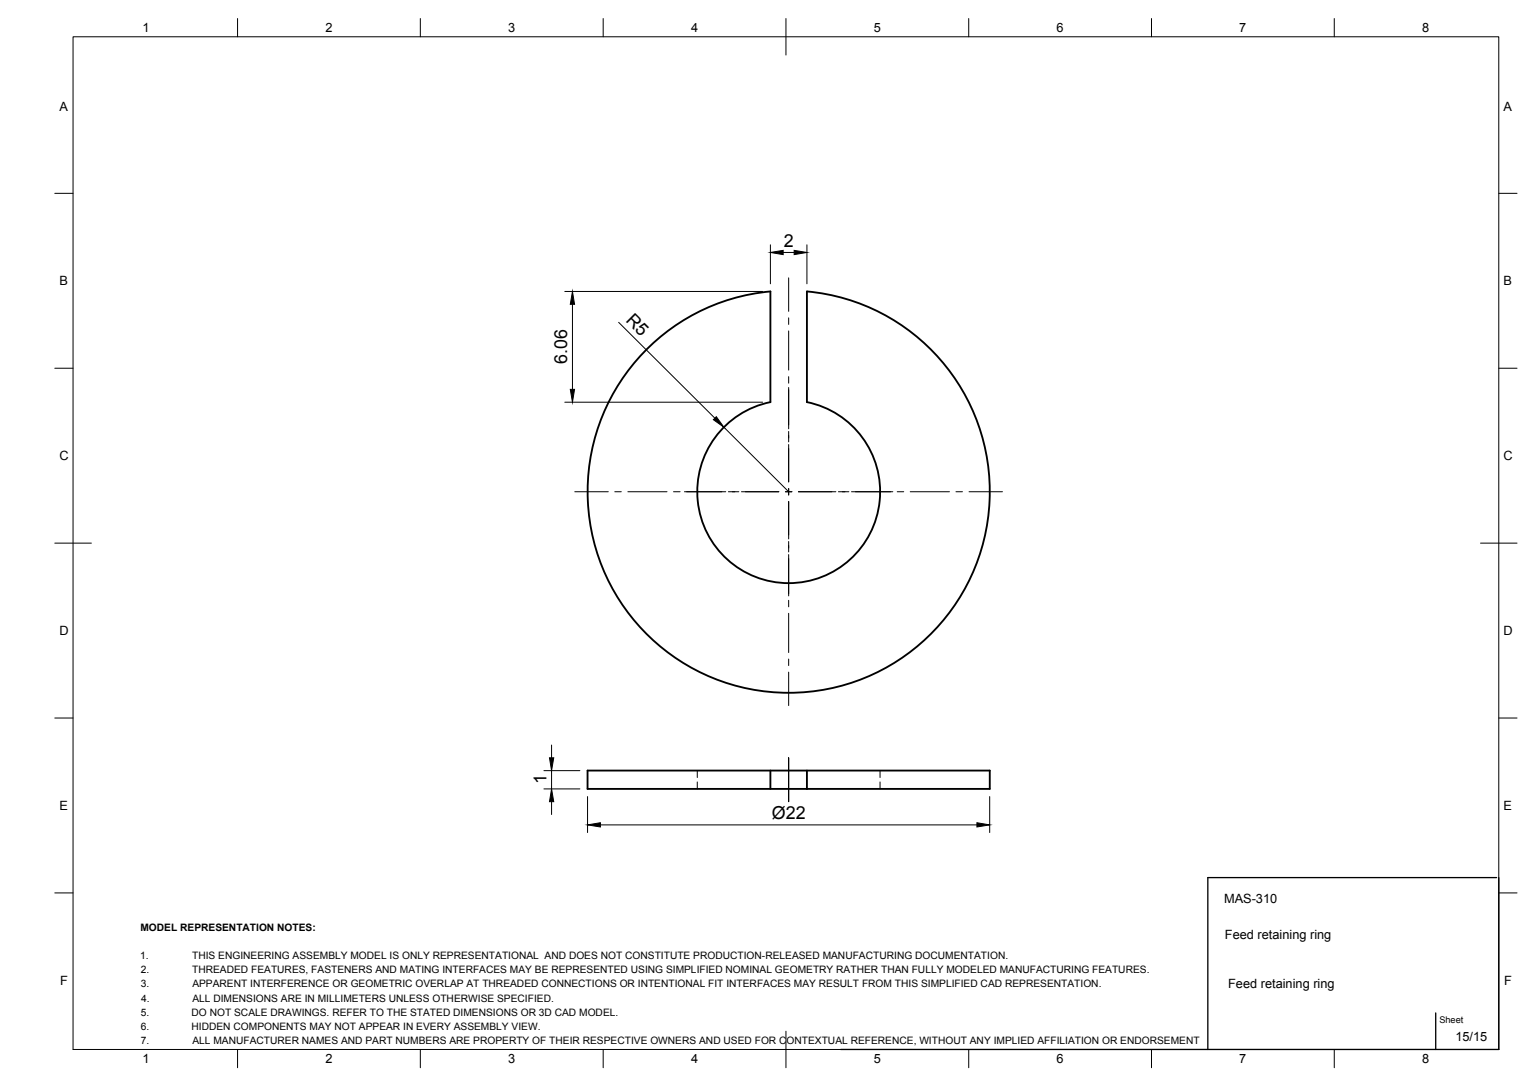
ISO-10303-21;
HEADER;
/* Generated by software containing ST-Developer
 * from STEP Tools, Inc. (www.steptools.com) 
 */

FILE_DESCRIPTION(
/* description */ ('Independent30mm screw-fed quill/spindle unit with16mm straight tool s
ocket, radial set screw, native reusable open ball bearings, retained 
inner/outer race stacks, keyed quill guide and M12x1.75 fine feed. Ext
ernal moving drive and tool not included. Ideal cage orbital links; in
dividual ball spin, force and preload not simulated. No drilling capac
ity, runout, speed, torque, load, life or machine safety rating.'),
/* implementation_level */ '2;1');

FILE_NAME(
/* name */ 'Feed retaining ring.step',
/* time_stamp */ '2026-11-08T18:59:42-08:00',
/* author */ (''),
/* organization */ (''),
/* preprocessor_version */ 'ST-DEVELOPER v20.2',
/* originating_system */ 'Autodesk Translation Framework v15.17.0.0',
/* authorisation */ '');

FILE_SCHEMA (('AUTOMOTIVE_DESIGN { 1 0 10303 214 3 1 1 }'));
ENDSEC;

DATA;
#10=MECHANICAL_DESIGN_GEOMETRIC_PRESENTATION_REPRESENTATION('',(#1601),#63898);
#1565=SHAPE_REPRESENTATION_RELATIONSHIP('SRR','None',#64004,#1583);
#1583=ADVANCED_BREP_SHAPE_REPRESENTATION('',(#1619),#63889);
#1601=STYLED_ITEM('',(#64099),#1619);
#1619=MANIFOLD_SOLID_BREP('Body1',#15487);
#2285=CYLINDRICAL_SURFACE('',#16526,5.);
#2286=CYLINDRICAL_SURFACE('',#16528,11.);
#2542=CIRCLE('',#16524,11.);
#2543=CIRCLE('',#16525,5.);
#2544=CIRCLE('',#16527,5.);
#2545=CIRCLE('',#16529,11.);
#3335=FACE_OUTER_BOUND('',#4236,.T.);
#3336=FACE_OUTER_BOUND('',#4237,.T.);
#3337=FACE_OUTER_BOUND('',#4238,.T.);
#3338=FACE_OUTER_BOUND('',#4239,.T.);
#3339=FACE_OUTER_BOUND('',#4240,.T.);
#3340=FACE_OUTER_BOUND('',#4241,.T.);
#4236=EDGE_LOOP('',(#13630,#13631,#13632,#13633));
#4237=EDGE_LOOP('',(#13634,#13635,#13636,#13637));
#4238=EDGE_LOOP('',(#13638,#13639,#13640,#13641));
#4239=EDGE_LOOP('',(#13642,#13643,#13644,#13645));
#4240=EDGE_LOOP('',(#13646,#13647,#13648,#13649));
#4241=EDGE_LOOP('',(#13650,#13651,#13652,#13653));
#5052=LINE('',#57567,#5815);
#5053=LINE('',#57569,#5816);
#5054=LINE('',#57571,#5817);
#5055=LINE('',#57572,#5818);
#5056=LINE('',#57576,#5819);
#5057=LINE('',#57578,#5820);
#5058=LINE('',#57580,#5821);
#5059=LINE('',#57581,#5822);
#5815=VECTOR('',#19142,10.);
#5816=VECTOR('',#19143,10.);
#5817=VECTOR('',#19144,10.);
#5818=VECTOR('',#19145,10.);
#5819=VECTOR('',#19148,10.);
#5820=VECTOR('',#19149,10.);
#5821=VECTOR('',#19150,10.);
#5822=VECTOR('',#19151,10.);
#7210=VERTEX_POINT('',#57565);
#7211=VERTEX_POINT('',#57566);
#7212=VERTEX_POINT('',#57568);
#7213=VERTEX_POINT('',#57570);
#7214=VERTEX_POINT('',#57574);
#7215=VERTEX_POINT('',#57575);
#7216=VERTEX_POINT('',#57577);
#7217=VERTEX_POINT('',#57579);
#9404=EDGE_CURVE('',#7210,#7211,#5052,.T.);
#9405=EDGE_CURVE('',#7212,#7210,#5053,.T.);
#9406=EDGE_CURVE('',#7213,#7212,#5054,.T.);
#9407=EDGE_CURVE('',#7211,#7213,#5055,.T.);
#9408=EDGE_CURVE('',#7214,#7215,#5056,.T.);
#9409=EDGE_CURVE('',#7216,#7214,#5057,.T.);
#9410=EDGE_CURVE('',#7217,#7216,#5058,.T.);
#9411=EDGE_CURVE('',#7215,#7217,#5059,.T.);
#9412=EDGE_CURVE('',#7212,#7217,#2542,.T.);
#9413=EDGE_CURVE('',#7215,#7210,#2543,.T.);
#9414=EDGE_CURVE('',#7214,#7211,#2544,.T.);
#9415=EDGE_CURVE('',#7213,#7216,#2545,.T.);
#13630=ORIENTED_EDGE('',*,*,#9404,.F.);
#13631=ORIENTED_EDGE('',*,*,#9405,.F.);
#13632=ORIENTED_EDGE('',*,*,#9406,.F.);
#13633=ORIENTED_EDGE('',*,*,#9407,.F.);
#13634=ORIENTED_EDGE('',*,*,#9408,.F.);
#13635=ORIENTED_EDGE('',*,*,#9409,.F.);
#13636=ORIENTED_EDGE('',*,*,#9410,.F.);
#13637=ORIENTED_EDGE('',*,*,#9411,.F.);
#13638=ORIENTED_EDGE('',*,*,#9411,.T.);
#13639=ORIENTED_EDGE('',*,*,#9412,.F.);
#13640=ORIENTED_EDGE('',*,*,#9405,.T.);
#13641=ORIENTED_EDGE('',*,*,#9413,.F.);
#13642=ORIENTED_EDGE('',*,*,#9408,.T.);
#13643=ORIENTED_EDGE('',*,*,#9413,.T.);
#13644=ORIENTED_EDGE('',*,*,#9404,.T.);
#13645=ORIENTED_EDGE('',*,*,#9414,.F.);
#13646=ORIENTED_EDGE('',*,*,#9410,.T.);
#13647=ORIENTED_EDGE('',*,*,#9415,.F.);
#13648=ORIENTED_EDGE('',*,*,#9406,.T.);
#13649=ORIENTED_EDGE('',*,*,#9412,.T.);
#13650=ORIENTED_EDGE('',*,*,#9409,.T.);
#13651=ORIENTED_EDGE('',*,*,#9414,.T.);
#13652=ORIENTED_EDGE('',*,*,#9407,.T.);
#13653=ORIENTED_EDGE('',*,*,#9415,.T.);
#14592=PLANE('',#16521);
#14593=PLANE('',#16522);
#14594=PLANE('',#16523);
#14595=PLANE('',#16530);
#15315=ADVANCED_FACE('',(#3335),#14592,.F.);
#15316=ADVANCED_FACE('',(#3336),#14593,.F.);
#15317=ADVANCED_FACE('',(#3337),#14594,.F.);
#15318=ADVANCED_FACE('',(#3338),#2285,.F.);
#15319=ADVANCED_FACE('',(#3339),#2286,.T.);
#15320=ADVANCED_FACE('',(#3340),#14595,.T.);
#15487=CLOSED_SHELL('',(#15315,#15316,#15317,#15318,#15319,#15320));
#16520=AXIS2_PLACEMENT_3D('',#57563,#19138,#19139);
#16521=AXIS2_PLACEMENT_3D('',#57564,#19140,#19141);
#16522=AXIS2_PLACEMENT_3D('',#57573,#19146,#19147);
#16523=AXIS2_PLACEMENT_3D('',#57582,#19152,#19153);
#16524=AXIS2_PLACEMENT_3D('',#57583,#19154,#19155);
#16525=AXIS2_PLACEMENT_3D('',#57584,#19156,#19157);
#16526=AXIS2_PLACEMENT_3D('',#57585,#19158,#19159);
#16527=AXIS2_PLACEMENT_3D('',#57586,#19160,#19161);
#16528=AXIS2_PLACEMENT_3D('',#57587,#19162,#19163);
#16529=AXIS2_PLACEMENT_3D('',#57588,#19164,#19165);
#16530=AXIS2_PLACEMENT_3D('',#57589,#19166,#19167);
#19138=DIRECTION('axis',(0.,0.,1.));
#19139=DIRECTION('refdir',(1.,0.,0.));
#19140=DIRECTION('center_axis',(-1.,0.,0.));
#19141=DIRECTION('ref_axis',(0.,1.,0.));
#19142=DIRECTION('',(0.,0.,1.));
#19143=DIRECTION('',(0.,-1.,0.));
#19144=DIRECTION('',(0.,0.,-1.));
#19145=DIRECTION('',(0.,1.,0.));
#19146=DIRECTION('center_axis',(1.,0.,0.));
#19147=DIRECTION('ref_axis',(0.,-1.,0.));
#19148=DIRECTION('',(0.,0.,-1.));
#19149=DIRECTION('',(0.,-1.,0.));
#19150=DIRECTION('',(0.,0.,1.));
#19151=DIRECTION('',(0.,1.,0.));
#19152=DIRECTION('center_axis',(0.,0.,1.));
#19153=DIRECTION('ref_axis',(1.,0.,0.));
#19154=DIRECTION('center_axis',(0.,0.,1.));
#19155=DIRECTION('ref_axis',(1.,0.,0.));
#19156=DIRECTION('center_axis',(0.,0.,-1.));
#19157=DIRECTION('ref_axis',(1.,0.,0.));
#19158=DIRECTION('center_axis',(0.,0.,1.));
#19159=DIRECTION('ref_axis',(6.12323399573677E-17,-1.,0.));
#19160=DIRECTION('center_axis',(0.,0.,-1.));
#19161=DIRECTION('ref_axis',(1.,0.,0.));
#19162=DIRECTION('center_axis',(0.,0.,1.));
#19163=DIRECTION('ref_axis',(6.12323399573677E-17,-1.,0.));
#19164=DIRECTION('center_axis',(0.,0.,1.));
#19165=DIRECTION('ref_axis',(1.,0.,0.));
#19166=DIRECTION('center_axis',(0.,0.,1.));
#19167=DIRECTION('ref_axis',(1.,0.,0.));
#57563=CARTESIAN_POINT('',(0.,0.,0.));
#57564=CARTESIAN_POINT('Origin',(-1.,0.,1.));
#57565=CARTESIAN_POINT('',(-1.,4.89897948556636,0.));
#57566=CARTESIAN_POINT('',(-1.,4.89897948556636,1.));
#57567=CARTESIAN_POINT('',(-1.,4.89897948556636,0.));
#57568=CARTESIAN_POINT('',(-1.,10.9544511501033,0.));
#57569=CARTESIAN_POINT('',(-1.,0.,0.));
#57570=CARTESIAN_POINT('',(-1.,10.9544511501033,1.));
#57571=CARTESIAN_POINT('',(-1.,10.9544511501033,0.));
#57572=CARTESIAN_POINT('',(-1.,0.,1.));
#57573=CARTESIAN_POINT('Origin',(1.,22.,1.));
#57574=CARTESIAN_POINT('',(1.,4.89897948556636,1.));
#57575=CARTESIAN_POINT('',(1.,4.89897948556636,0.));
#57576=CARTESIAN_POINT('',(1.,4.89897948556636,0.));
#57577=CARTESIAN_POINT('',(1.,10.9544511501033,1.));
#57578=CARTESIAN_POINT('',(1.,11.,1.));
#57579=CARTESIAN_POINT('',(1.,10.9544511501033,0.));
#57580=CARTESIAN_POINT('',(1.,10.9544511501033,0.));
#57581=CARTESIAN_POINT('',(1.,11.,0.));
#57582=CARTESIAN_POINT('Origin',(0.,0.,0.));
#57583=CARTESIAN_POINT('Origin',(0.,0.,0.));
#57584=CARTESIAN_POINT('Origin',(0.,0.,0.));
#57585=CARTESIAN_POINT('Origin',(0.,0.,0.));
#57586=CARTESIAN_POINT('Origin',(0.,0.,1.));
#57587=CARTESIAN_POINT('Origin',(0.,0.,0.));
#57588=CARTESIAN_POINT('Origin',(0.,0.,1.));
#57589=CARTESIAN_POINT('Origin',(0.,0.,1.));
#63869=UNCERTAINTY_MEASURE_WITH_UNIT(LENGTH_MEASURE(0.01),#63899,
'DISTANCE_ACCURACY_VALUE',
'Maximum model space distance between geometric entities at asserted c
onnectivities');
#63878=UNCERTAINTY_MEASURE_WITH_UNIT(LENGTH_MEASURE(0.01),#63899,
'DISTANCE_ACCURACY_VALUE',
'Maximum model space distance between geometric entities at asserted c
onnectivities');
#63889=(
GEOMETRIC_REPRESENTATION_CONTEXT(3)
GLOBAL_UNCERTAINTY_ASSIGNED_CONTEXT((#63869))
GLOBAL_UNIT_ASSIGNED_CONTEXT((#63899,#63901,#63902))
REPRESENTATION_CONTEXT('','3D')
);
#63898=(
GEOMETRIC_REPRESENTATION_CONTEXT(3)
GLOBAL_UNCERTAINTY_ASSIGNED_CONTEXT((#63878))
GLOBAL_UNIT_ASSIGNED_CONTEXT((#63899,#63901,#63902))
REPRESENTATION_CONTEXT('','3D')
);
#63899=(
LENGTH_UNIT()
NAMED_UNIT(*)
SI_UNIT(.MILLI.,.METRE.)
);
#63901=(
NAMED_UNIT(*)
PLANE_ANGLE_UNIT()
SI_UNIT($,.RADIAN.)
);
#63902=(
NAMED_UNIT(*)
SI_UNIT($,.STERADIAN.)
SOLID_ANGLE_UNIT()
);
#63913=SHAPE_DEFINITION_REPRESENTATION(#63932,#64004);
#63932=PRODUCT_DEFINITION_SHAPE('',$,#64024);
#64004=SHAPE_REPRESENTATION('',(#16520),#63889);
#64013=PRODUCT_DEFINITION_CONTEXT('part definition',#64072,'design');
#64024=PRODUCT_DEFINITION('Feed retaining ring','Feed retaining ring',#64043,
#64013);
#64043=PRODUCT_DEFINITION_FORMATION('',$,#64084);
#64072=APPLICATION_CONTEXT(
'Core Data for Automotive Mechanical Design Process');
#64073=PRODUCT_CONTEXT('part definition',#64072,'mechanical');
#64084=PRODUCT('Feed retaining ring','Feed retaining ring',$,(#64073));
#64099=PRESENTATION_STYLE_ASSIGNMENT((#64112));
#64112=SURFACE_STYLE_USAGE(.BOTH.,#64125);
#64125=SURFACE_SIDE_STYLE('',(#64138));
#64138=SURFACE_STYLE_FILL_AREA(#64151);
#64151=FILL_AREA_STYLE('Dark gray',(#64164));
#64164=FILL_AREA_STYLE_COLOUR('Dark gray',#64177);
#64177=COLOUR_RGB('Dark gray',0.250980392156863,0.282352941176471,0.32156862745098);
ENDSEC;
END-ISO-10303-21;
